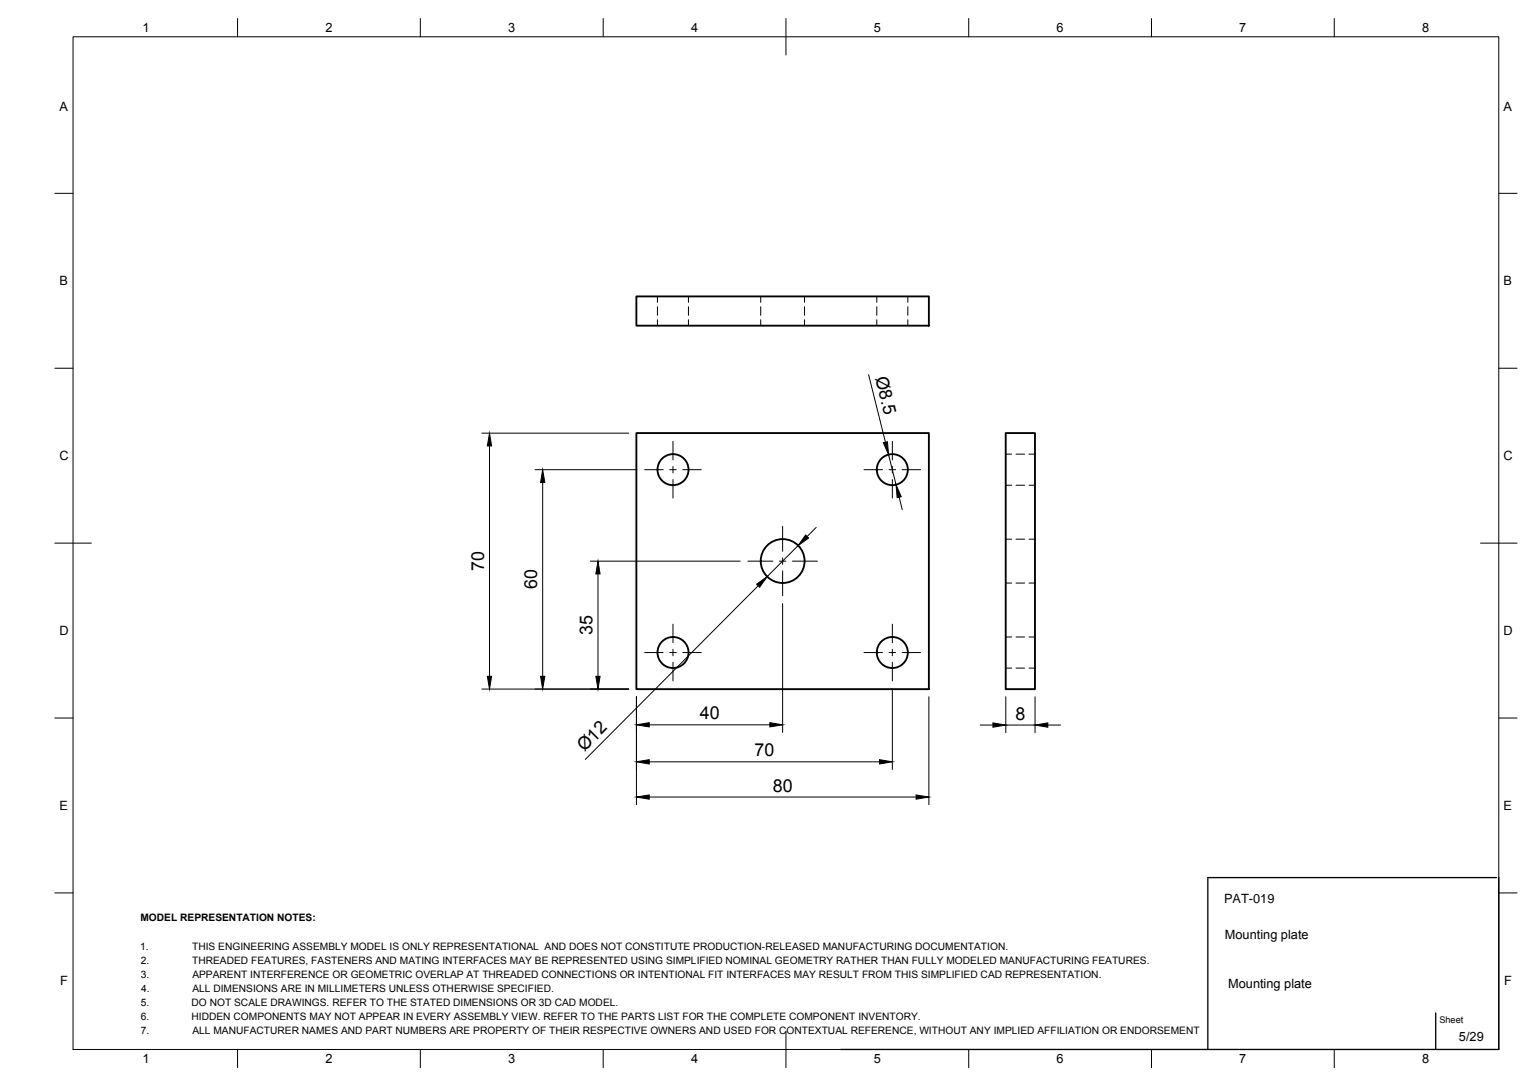
ISO-10303-21;
HEADER;
/* Generated by software containing ST-Developer
 * from STEP Tools, Inc. (www.steptools.com) 
 */

FILE_DESCRIPTION(
/* description */ ('Caster wheel assembly'),
/* implementation_level */ '2;1');

FILE_NAME(
/* name */ 'Mounting plate.step',
/* time_stamp */ '2026-10-28T03:23:56-07:00',
/* author */ (''),
/* organization */ (''),
/* preprocessor_version */ 'ST-DEVELOPER v20.2',
/* originating_system */ 'Autodesk Translation Framework v15.17.0.0',
/* authorisation */ '');

FILE_SCHEMA (('AUTOMOTIVE_DESIGN { 1 0 10303 214 3 1 1 }'));
ENDSEC;

DATA;
#10=MECHANICAL_DESIGN_GEOMETRIC_PRESENTATION_REPRESENTATION('',(#222),#5385);
#178=SHAPE_REPRESENTATION_RELATIONSHIP('SRR','None',#5473,#200);
#200=ADVANCED_BREP_SHAPE_REPRESENTATION('',(#252),#5360);
#222=STYLED_ITEM('',(#5658),#252);
#252=MANIFOLD_SOLID_BREP('Body1',#2649);
#281=FACE_BOUND('',#599,.T.);
#282=FACE_BOUND('',#600,.T.);
#283=FACE_BOUND('',#601,.T.);
#284=FACE_BOUND('',#602,.T.);
#285=FACE_BOUND('',#603,.T.);
#286=FACE_BOUND('',#605,.T.);
#287=FACE_BOUND('',#606,.T.);
#288=FACE_BOUND('',#607,.T.);
#289=FACE_BOUND('',#608,.T.);
#290=FACE_BOUND('',#609,.T.);
#333=PLANE('',#2941);
#334=PLANE('',#2942);
#335=PLANE('',#2943);
#336=PLANE('',#2944);
#337=PLANE('',#2945);
#338=PLANE('',#2946);
#421=FACE_OUTER_BOUND('',#589,.T.);
#422=FACE_OUTER_BOUND('',#590,.T.);
#423=FACE_OUTER_BOUND('',#591,.T.);
#424=FACE_OUTER_BOUND('',#592,.T.);
#425=FACE_OUTER_BOUND('',#593,.T.);
#426=FACE_OUTER_BOUND('',#594,.T.);
#427=FACE_OUTER_BOUND('',#595,.T.);
#428=FACE_OUTER_BOUND('',#596,.T.);
#429=FACE_OUTER_BOUND('',#597,.T.);
#430=FACE_OUTER_BOUND('',#598,.T.);
#431=FACE_OUTER_BOUND('',#604,.T.);
#589=EDGE_LOOP('',(#1782,#1783,#1784,#1785));
#590=EDGE_LOOP('',(#1786,#1787,#1788,#1789));
#591=EDGE_LOOP('',(#1790,#1791,#1792,#1793));
#592=EDGE_LOOP('',(#1794,#1795,#1796,#1797));
#593=EDGE_LOOP('',(#1798,#1799,#1800,#1801));
#594=EDGE_LOOP('',(#1802,#1803,#1804,#1805));
#595=EDGE_LOOP('',(#1806,#1807,#1808,#1809));
#596=EDGE_LOOP('',(#1810,#1811,#1812,#1813));
#597=EDGE_LOOP('',(#1814,#1815,#1816,#1817));
#598=EDGE_LOOP('',(#1818,#1819,#1820,#1821));
#599=EDGE_LOOP('',(#1822));
#600=EDGE_LOOP('',(#1823));
#601=EDGE_LOOP('',(#1824));
#602=EDGE_LOOP('',(#1825));
#603=EDGE_LOOP('',(#1826));
#604=EDGE_LOOP('',(#1827,#1828,#1829,#1830));
#605=EDGE_LOOP('',(#1831));
#606=EDGE_LOOP('',(#1832));
#607=EDGE_LOOP('',(#1833));
#608=EDGE_LOOP('',(#1834));
#609=EDGE_LOOP('',(#1835));
#809=LINE('',#4207,#943);
#810=LINE('',#4213,#944);
#811=LINE('',#4219,#945);
#812=LINE('',#4225,#946);
#813=LINE('',#4231,#947);
#814=LINE('',#4236,#948);
#815=LINE('',#4238,#949);
#816=LINE('',#4240,#950);
#817=LINE('',#4241,#951);
#818=LINE('',#4244,#952);
#819=LINE('',#4246,#953);
#820=LINE('',#4247,#954);
#821=LINE('',#4250,#955);
#822=LINE('',#4252,#956);
#823=LINE('',#4253,#957);
#824=LINE('',#4255,#958);
#825=LINE('',#4256,#959);
#943=VECTOR('',#3314,0.6);
#944=VECTOR('',#3321,0.425);
#945=VECTOR('',#3328,0.425);
#946=VECTOR('',#3335,0.425);
#947=VECTOR('',#3342,0.425);
#948=VECTOR('',#3347,1.);
#949=VECTOR('',#3348,1.);
#950=VECTOR('',#3349,1.);
#951=VECTOR('',#3350,1.);
#952=VECTOR('',#3353,1.);
#953=VECTOR('',#3354,1.);
#954=VECTOR('',#3355,1.);
#955=VECTOR('',#3358,1.);
#956=VECTOR('',#3359,1.);
#957=VECTOR('',#3360,1.);
#958=VECTOR('',#3363,1.);
#959=VECTOR('',#3364,1.);
#1077=CIRCLE('',#2927,0.6);
#1078=CIRCLE('',#2928,0.6);
#1079=CIRCLE('',#2930,0.425);
#1080=CIRCLE('',#2931,0.425);
#1081=CIRCLE('',#2933,0.425);
#1082=CIRCLE('',#2934,0.425);
#1083=CIRCLE('',#2936,0.425);
#1084=CIRCLE('',#2937,0.425);
#1085=CIRCLE('',#2939,0.425);
#1086=CIRCLE('',#2940,0.425);
#1236=VERTEX_POINT('',#4204);
#1237=VERTEX_POINT('',#4206);
#1238=VERTEX_POINT('',#4210);
#1239=VERTEX_POINT('',#4212);
#1240=VERTEX_POINT('',#4216);
#1241=VERTEX_POINT('',#4218);
#1242=VERTEX_POINT('',#4222);
#1243=VERTEX_POINT('',#4224);
#1244=VERTEX_POINT('',#4228);
#1245=VERTEX_POINT('',#4230);
#1246=VERTEX_POINT('',#4234);
#1247=VERTEX_POINT('',#4235);
#1248=VERTEX_POINT('',#4237);
#1249=VERTEX_POINT('',#4239);
#1250=VERTEX_POINT('',#4243);
#1251=VERTEX_POINT('',#4245);
#1252=VERTEX_POINT('',#4249);
#1253=VERTEX_POINT('',#4251);
#1459=EDGE_CURVE('',#1236,#1236,#1077,.T.);
#1460=EDGE_CURVE('',#1236,#1237,#809,.T.);
#1461=EDGE_CURVE('',#1237,#1237,#1078,.T.);
#1462=EDGE_CURVE('',#1238,#1238,#1079,.T.);
#1463=EDGE_CURVE('',#1238,#1239,#810,.T.);
#1464=EDGE_CURVE('',#1239,#1239,#1080,.T.);
#1465=EDGE_CURVE('',#1240,#1240,#1081,.T.);
#1466=EDGE_CURVE('',#1240,#1241,#811,.T.);
#1467=EDGE_CURVE('',#1241,#1241,#1082,.T.);
#1468=EDGE_CURVE('',#1242,#1242,#1083,.T.);
#1469=EDGE_CURVE('',#1242,#1243,#812,.T.);
#1470=EDGE_CURVE('',#1243,#1243,#1084,.T.);
#1471=EDGE_CURVE('',#1244,#1244,#1085,.T.);
#1472=EDGE_CURVE('',#1244,#1245,#813,.T.);
#1473=EDGE_CURVE('',#1245,#1245,#1086,.T.);
#1474=EDGE_CURVE('',#1246,#1247,#814,.T.);
#1475=EDGE_CURVE('',#1247,#1248,#815,.T.);
#1476=EDGE_CURVE('',#1249,#1248,#816,.T.);
#1477=EDGE_CURVE('',#1246,#1249,#817,.T.);
#1478=EDGE_CURVE('',#1250,#1246,#818,.T.);
#1479=EDGE_CURVE('',#1251,#1249,#819,.T.);
#1480=EDGE_CURVE('',#1250,#1251,#820,.T.);
#1481=EDGE_CURVE('',#1252,#1250,#821,.T.);
#1482=EDGE_CURVE('',#1253,#1251,#822,.T.);
#1483=EDGE_CURVE('',#1252,#1253,#823,.T.);
#1484=EDGE_CURVE('',#1247,#1252,#824,.T.);
#1485=EDGE_CURVE('',#1248,#1253,#825,.T.);
#1782=ORIENTED_EDGE('',*,*,#1459,.F.);
#1783=ORIENTED_EDGE('',*,*,#1460,.T.);
#1784=ORIENTED_EDGE('',*,*,#1461,.F.);
#1785=ORIENTED_EDGE('',*,*,#1460,.F.);
#1786=ORIENTED_EDGE('',*,*,#1462,.F.);
#1787=ORIENTED_EDGE('',*,*,#1463,.T.);
#1788=ORIENTED_EDGE('',*,*,#1464,.F.);
#1789=ORIENTED_EDGE('',*,*,#1463,.F.);
#1790=ORIENTED_EDGE('',*,*,#1465,.F.);
#1791=ORIENTED_EDGE('',*,*,#1466,.T.);
#1792=ORIENTED_EDGE('',*,*,#1467,.F.);
#1793=ORIENTED_EDGE('',*,*,#1466,.F.);
#1794=ORIENTED_EDGE('',*,*,#1468,.F.);
#1795=ORIENTED_EDGE('',*,*,#1469,.T.);
#1796=ORIENTED_EDGE('',*,*,#1470,.F.);
#1797=ORIENTED_EDGE('',*,*,#1469,.F.);
#1798=ORIENTED_EDGE('',*,*,#1471,.F.);
#1799=ORIENTED_EDGE('',*,*,#1472,.T.);
#1800=ORIENTED_EDGE('',*,*,#1473,.F.);
#1801=ORIENTED_EDGE('',*,*,#1472,.F.);
#1802=ORIENTED_EDGE('',*,*,#1474,.T.);
#1803=ORIENTED_EDGE('',*,*,#1475,.T.);
#1804=ORIENTED_EDGE('',*,*,#1476,.F.);
#1805=ORIENTED_EDGE('',*,*,#1477,.F.);
#1806=ORIENTED_EDGE('',*,*,#1478,.T.);
#1807=ORIENTED_EDGE('',*,*,#1477,.T.);
#1808=ORIENTED_EDGE('',*,*,#1479,.F.);
#1809=ORIENTED_EDGE('',*,*,#1480,.F.);
#1810=ORIENTED_EDGE('',*,*,#1481,.T.);
#1811=ORIENTED_EDGE('',*,*,#1480,.T.);
#1812=ORIENTED_EDGE('',*,*,#1482,.F.);
#1813=ORIENTED_EDGE('',*,*,#1483,.F.);
#1814=ORIENTED_EDGE('',*,*,#1484,.T.);
#1815=ORIENTED_EDGE('',*,*,#1483,.T.);
#1816=ORIENTED_EDGE('',*,*,#1485,.F.);
#1817=ORIENTED_EDGE('',*,*,#1475,.F.);
#1818=ORIENTED_EDGE('',*,*,#1485,.T.);
#1819=ORIENTED_EDGE('',*,*,#1482,.T.);
#1820=ORIENTED_EDGE('',*,*,#1479,.T.);
#1821=ORIENTED_EDGE('',*,*,#1476,.T.);
#1822=ORIENTED_EDGE('',*,*,#1461,.T.);
#1823=ORIENTED_EDGE('',*,*,#1464,.T.);
#1824=ORIENTED_EDGE('',*,*,#1467,.T.);
#1825=ORIENTED_EDGE('',*,*,#1470,.T.);
#1826=ORIENTED_EDGE('',*,*,#1473,.T.);
#1827=ORIENTED_EDGE('',*,*,#1484,.F.);
#1828=ORIENTED_EDGE('',*,*,#1474,.F.);
#1829=ORIENTED_EDGE('',*,*,#1478,.F.);
#1830=ORIENTED_EDGE('',*,*,#1481,.F.);
#1831=ORIENTED_EDGE('',*,*,#1459,.T.);
#1832=ORIENTED_EDGE('',*,*,#1462,.T.);
#1833=ORIENTED_EDGE('',*,*,#1465,.T.);
#1834=ORIENTED_EDGE('',*,*,#1468,.T.);
#1835=ORIENTED_EDGE('',*,*,#1471,.T.);
#2428=CYLINDRICAL_SURFACE('',#2926,0.6);
#2429=CYLINDRICAL_SURFACE('',#2929,0.425);
#2430=CYLINDRICAL_SURFACE('',#2932,0.425);
#2431=CYLINDRICAL_SURFACE('',#2935,0.425);
#2432=CYLINDRICAL_SURFACE('',#2938,0.425);
#2481=ADVANCED_FACE('',(#421),#2428,.F.);
#2482=ADVANCED_FACE('',(#422),#2429,.F.);
#2483=ADVANCED_FACE('',(#423),#2430,.F.);
#2484=ADVANCED_FACE('',(#424),#2431,.F.);
#2485=ADVANCED_FACE('',(#425),#2432,.F.);
#2486=ADVANCED_FACE('',(#426),#333,.T.);
#2487=ADVANCED_FACE('',(#427),#334,.T.);
#2488=ADVANCED_FACE('',(#428),#335,.T.);
#2489=ADVANCED_FACE('',(#429),#336,.T.);
#2490=ADVANCED_FACE('',(#430,#281,#282,#283,#284,#285),#337,.T.);
#2491=ADVANCED_FACE('',(#431,#286,#287,#288,#289,#290),#338,.F.);
#2649=CLOSED_SHELL('',(#2481,#2482,#2483,#2484,#2485,#2486,#2487,#2488,
#2489,#2490,#2491));
#2925=AXIS2_PLACEMENT_3D('',#4202,#3308,#3309);
#2926=AXIS2_PLACEMENT_3D('',#4203,#3310,#3311);
#2927=AXIS2_PLACEMENT_3D('',#4205,#3312,#3313);
#2928=AXIS2_PLACEMENT_3D('',#4208,#3315,#3316);
#2929=AXIS2_PLACEMENT_3D('',#4209,#3317,#3318);
#2930=AXIS2_PLACEMENT_3D('',#4211,#3319,#3320);
#2931=AXIS2_PLACEMENT_3D('',#4214,#3322,#3323);
#2932=AXIS2_PLACEMENT_3D('',#4215,#3324,#3325);
#2933=AXIS2_PLACEMENT_3D('',#4217,#3326,#3327);
#2934=AXIS2_PLACEMENT_3D('',#4220,#3329,#3330);
#2935=AXIS2_PLACEMENT_3D('',#4221,#3331,#3332);
#2936=AXIS2_PLACEMENT_3D('',#4223,#3333,#3334);
#2937=AXIS2_PLACEMENT_3D('',#4226,#3336,#3337);
#2938=AXIS2_PLACEMENT_3D('',#4227,#3338,#3339);
#2939=AXIS2_PLACEMENT_3D('',#4229,#3340,#3341);
#2940=AXIS2_PLACEMENT_3D('',#4232,#3343,#3344);
#2941=AXIS2_PLACEMENT_3D('',#4233,#3345,#3346);
#2942=AXIS2_PLACEMENT_3D('',#4242,#3351,#3352);
#2943=AXIS2_PLACEMENT_3D('',#4248,#3356,#3357);
#2944=AXIS2_PLACEMENT_3D('',#4254,#3361,#3362);
#2945=AXIS2_PLACEMENT_3D('',#4257,#3365,#3366);
#2946=AXIS2_PLACEMENT_3D('',#4258,#3367,#3368);
#3308=DIRECTION('axis',(0.,0.,1.));
#3309=DIRECTION('refdir',(1.,0.,0.));
#3310=DIRECTION('center_axis',(0.,0.,1.));
#3311=DIRECTION('ref_axis',(1.,0.,0.));
#3312=DIRECTION('center_axis',(0.,0.,1.));
#3313=DIRECTION('ref_axis',(1.,0.,0.));
#3314=DIRECTION('',(0.,0.,1.));
#3315=DIRECTION('center_axis',(0.,0.,-1.));
#3316=DIRECTION('ref_axis',(1.,0.,0.));
#3317=DIRECTION('center_axis',(0.,0.,1.));
#3318=DIRECTION('ref_axis',(1.,0.,0.));
#3319=DIRECTION('center_axis',(0.,0.,1.));
#3320=DIRECTION('ref_axis',(1.,0.,0.));
#3321=DIRECTION('',(0.,0.,1.));
#3322=DIRECTION('center_axis',(0.,0.,-1.));
#3323=DIRECTION('ref_axis',(1.,0.,0.));
#3324=DIRECTION('center_axis',(0.,0.,1.));
#3325=DIRECTION('ref_axis',(1.,0.,0.));
#3326=DIRECTION('center_axis',(0.,0.,1.));
#3327=DIRECTION('ref_axis',(1.,0.,0.));
#3328=DIRECTION('',(0.,0.,1.));
#3329=DIRECTION('center_axis',(0.,0.,-1.));
#3330=DIRECTION('ref_axis',(1.,0.,0.));
#3331=DIRECTION('center_axis',(0.,0.,1.));
#3332=DIRECTION('ref_axis',(1.,0.,0.));
#3333=DIRECTION('center_axis',(0.,0.,1.));
#3334=DIRECTION('ref_axis',(1.,0.,0.));
#3335=DIRECTION('',(0.,0.,1.));
#3336=DIRECTION('center_axis',(0.,0.,-1.));
#3337=DIRECTION('ref_axis',(1.,0.,0.));
#3338=DIRECTION('center_axis',(0.,0.,1.));
#3339=DIRECTION('ref_axis',(1.,0.,0.));
#3340=DIRECTION('center_axis',(0.,0.,1.));
#3341=DIRECTION('ref_axis',(1.,0.,0.));
#3342=DIRECTION('',(0.,0.,1.));
#3343=DIRECTION('center_axis',(0.,0.,-1.));
#3344=DIRECTION('ref_axis',(1.,0.,0.));
#3345=DIRECTION('center_axis',(0.,1.,0.));
#3346=DIRECTION('ref_axis',(-1.,0.,0.));
#3347=DIRECTION('',(-1.,0.,0.));
#3348=DIRECTION('',(0.,0.,1.));
#3349=DIRECTION('',(-1.,0.,0.));
#3350=DIRECTION('',(0.,0.,1.));
#3351=DIRECTION('center_axis',(1.,0.,0.));
#3352=DIRECTION('ref_axis',(0.,1.,0.));
#3353=DIRECTION('',(0.,1.,0.));
#3354=DIRECTION('',(0.,1.,0.));
#3355=DIRECTION('',(0.,0.,1.));
#3356=DIRECTION('center_axis',(0.,-1.,0.));
#3357=DIRECTION('ref_axis',(1.,0.,0.));
#3358=DIRECTION('',(1.,0.,0.));
#3359=DIRECTION('',(1.,0.,0.));
#3360=DIRECTION('',(0.,0.,1.));
#3361=DIRECTION('center_axis',(-1.,0.,0.));
#3362=DIRECTION('ref_axis',(0.,-1.,0.));
#3363=DIRECTION('',(0.,-1.,0.));
#3364=DIRECTION('',(0.,-1.,0.));
#3365=DIRECTION('center_axis',(0.,0.,1.));
#3366=DIRECTION('ref_axis',(1.,0.,0.));
#3367=DIRECTION('center_axis',(0.,0.,1.));
#3368=DIRECTION('ref_axis',(1.,0.,0.));
#4202=CARTESIAN_POINT('',(0.,0.,0.));
#4203=CARTESIAN_POINT('Origin',(-2.,0.,9.6));
#4204=CARTESIAN_POINT('',(-2.6,-7.34788079488412E-17,9.7));
#4205=CARTESIAN_POINT('Origin',(-2.,0.,9.7));
#4206=CARTESIAN_POINT('',(-2.6,7.34788079488412E-17,10.5));
#4207=CARTESIAN_POINT('',(-2.6,-7.34788079488412E-17,9.6));
#4208=CARTESIAN_POINT('Origin',(-2.,0.,10.5));
#4209=CARTESIAN_POINT('Origin',(1.,-2.5,9.6));
#4210=CARTESIAN_POINT('',(0.575,-2.5,9.7));
#4211=CARTESIAN_POINT('Origin',(1.,-2.5,9.7));
#4212=CARTESIAN_POINT('',(0.575,-2.5,10.5));
#4213=CARTESIAN_POINT('',(0.575,-2.5,9.6));
#4214=CARTESIAN_POINT('Origin',(1.,-2.5,10.5));
#4215=CARTESIAN_POINT('Origin',(-5.,2.5,9.6));
#4216=CARTESIAN_POINT('',(-5.425,2.5,9.7));
#4217=CARTESIAN_POINT('Origin',(-5.,2.5,9.7));
#4218=CARTESIAN_POINT('',(-5.425,2.5,10.5));
#4219=CARTESIAN_POINT('',(-5.425,2.5,9.6));
#4220=CARTESIAN_POINT('Origin',(-5.,2.5,10.5));
#4221=CARTESIAN_POINT('Origin',(-5.,-2.5,9.6));
#4222=CARTESIAN_POINT('',(-5.425,-2.5,9.7));
#4223=CARTESIAN_POINT('Origin',(-5.,-2.5,9.7));
#4224=CARTESIAN_POINT('',(-5.425,-2.5,10.5));
#4225=CARTESIAN_POINT('',(-5.425,-2.5,9.6));
#4226=CARTESIAN_POINT('Origin',(-5.,-2.5,10.5));
#4227=CARTESIAN_POINT('Origin',(1.,2.5,9.6));
#4228=CARTESIAN_POINT('',(0.575,2.5,9.7));
#4229=CARTESIAN_POINT('Origin',(1.,2.5,9.7));
#4230=CARTESIAN_POINT('',(0.575,2.5,10.5));
#4231=CARTESIAN_POINT('',(0.575,2.5,9.6));
#4232=CARTESIAN_POINT('Origin',(1.,2.5,10.5));
#4233=CARTESIAN_POINT('Origin',(2.,3.5,9.7));
#4234=CARTESIAN_POINT('',(2.,3.5,9.7));
#4235=CARTESIAN_POINT('',(-6.,3.5,9.7));
#4236=CARTESIAN_POINT('',(2.,3.5,9.7));
#4237=CARTESIAN_POINT('',(-6.,3.5,10.5));
#4238=CARTESIAN_POINT('',(-6.,3.5,9.7));
#4239=CARTESIAN_POINT('',(2.,3.5,10.5));
#4240=CARTESIAN_POINT('',(2.,3.5,10.5));
#4241=CARTESIAN_POINT('',(2.,3.5,9.7));
#4242=CARTESIAN_POINT('Origin',(2.,-3.5,9.7));
#4243=CARTESIAN_POINT('',(2.,-3.5,9.7));
#4244=CARTESIAN_POINT('',(2.,-3.5,9.7));
#4245=CARTESIAN_POINT('',(2.,-3.5,10.5));
#4246=CARTESIAN_POINT('',(2.,-3.5,10.5));
#4247=CARTESIAN_POINT('',(2.,-3.5,9.7));
#4248=CARTESIAN_POINT('Origin',(-6.,-3.5,9.7));
#4249=CARTESIAN_POINT('',(-6.,-3.5,9.7));
#4250=CARTESIAN_POINT('',(-6.,-3.5,9.7));
#4251=CARTESIAN_POINT('',(-6.,-3.5,10.5));
#4252=CARTESIAN_POINT('',(-6.,-3.5,10.5));
#4253=CARTESIAN_POINT('',(-6.,-3.5,9.7));
#4254=CARTESIAN_POINT('Origin',(-6.,3.5,9.7));
#4255=CARTESIAN_POINT('',(-6.,3.5,9.7));
#4256=CARTESIAN_POINT('',(-6.,3.5,10.5));
#4257=CARTESIAN_POINT('Origin',(-2.,0.,10.5));
#4258=CARTESIAN_POINT('Origin',(-2.,0.,9.7));
#5332=UNCERTAINTY_MEASURE_WITH_UNIT(LENGTH_MEASURE(0.001),#5386,
'DISTANCE_ACCURACY_VALUE',
'Maximum model space distance between geometric entities at asserted c
onnectivities');
#5357=UNCERTAINTY_MEASURE_WITH_UNIT(LENGTH_MEASURE(0.001),#5386,
'DISTANCE_ACCURACY_VALUE',
'Maximum model space distance between geometric entities at asserted c
onnectivities');
#5360=(
GEOMETRIC_REPRESENTATION_CONTEXT(3)
GLOBAL_UNCERTAINTY_ASSIGNED_CONTEXT((#5332))
GLOBAL_UNIT_ASSIGNED_CONTEXT((#5386,#5388,#5389))
REPRESENTATION_CONTEXT('','3D')
);
#5385=(
GEOMETRIC_REPRESENTATION_CONTEXT(3)
GLOBAL_UNCERTAINTY_ASSIGNED_CONTEXT((#5357))
GLOBAL_UNIT_ASSIGNED_CONTEXT((#5386,#5388,#5389))
REPRESENTATION_CONTEXT('','3D')
);
#5386=(
LENGTH_UNIT()
NAMED_UNIT(*)
SI_UNIT(.CENTI.,.METRE.)
);
#5388=(
NAMED_UNIT(*)
PLANE_ANGLE_UNIT()
SI_UNIT($,.RADIAN.)
);
#5389=(
NAMED_UNIT(*)
SI_UNIT($,.STERADIAN.)
SOLID_ANGLE_UNIT()
);
#5392=SHAPE_DEFINITION_REPRESENTATION(#5419,#5473);
#5419=PRODUCT_DEFINITION_SHAPE('',$,#5501);
#5473=SHAPE_REPRESENTATION('',(#2925),#5360);
#5498=PRODUCT_DEFINITION_CONTEXT('part definition',#5581,'design');
#5501=PRODUCT_DEFINITION('Mounting plate','Mounting plate',#5528,#5498);
#5528=PRODUCT_DEFINITION_FORMATION('',$,#5585);
#5581=APPLICATION_CONTEXT(
'Core Data for Automotive Mechanical Design Process');
#5582=PRODUCT_CONTEXT('part definition',#5581,'mechanical');
#5585=PRODUCT('Mounting plate','Mounting plate','Mounting plate',(#5582));
#5652=COLOUR_RGB('Light Blue',0.38,0.62,0.78);
#5653=FILL_AREA_STYLE_COLOUR('',#5652);
#5654=FILL_AREA_STYLE('',(#5653));
#5655=SURFACE_STYLE_FILL_AREA(#5654);
#5656=SURFACE_SIDE_STYLE('',(#5655));
#5657=SURFACE_STYLE_USAGE(.BOTH.,#5656);
#5658=PRESENTATION_STYLE_ASSIGNMENT((#5657));
ENDSEC;
END-ISO-10303-21;
